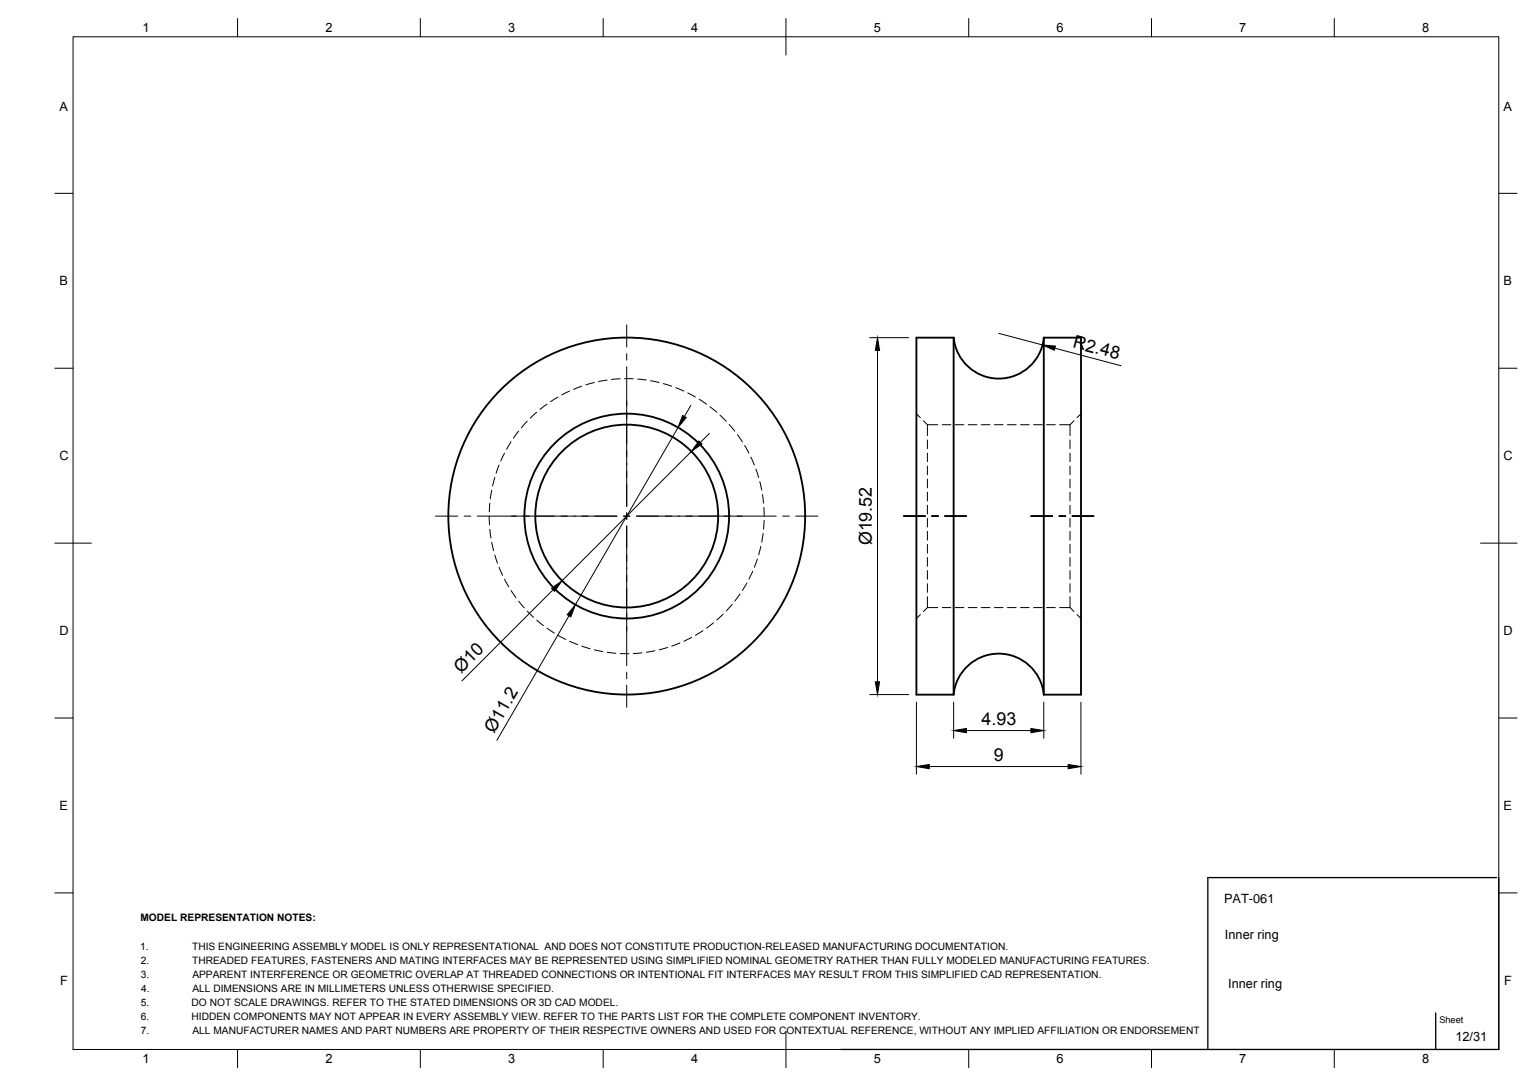
ISO-10303-21;
HEADER;
/* Generated by software containing ST-Developer
 * from STEP Tools, Inc. (www.steptools.com) 
 */

FILE_DESCRIPTION(
/* description */ ('Compact intermittent indexer'),
/* implementation_level */ '2;1');

FILE_NAME(
/* name */ 'Inner ring.step',
/* time_stamp */ '2026-10-29T16:32:17-07:00',
/* author */ (''),
/* organization */ (''),
/* preprocessor_version */ 'ST-DEVELOPER v20.2',
/* originating_system */ 'Autodesk Translation Framework v15.17.0.0',
/* authorisation */ '');

FILE_SCHEMA (('AUTOMOTIVE_DESIGN { 1 0 10303 214 3 1 1 }'));
ENDSEC;

DATA;
#10=MECHANICAL_DESIGN_GEOMETRIC_PRESENTATION_REPRESENTATION('',(#263),#10837);
#191=TOROIDAL_SURFACE('',#6190,1.,0.247676);
#199=CONICAL_SURFACE('',#6201,0.53,0.785398163397448);
#200=CONICAL_SURFACE('',#6208,0.53,0.785398163397448);
#215=SHAPE_REPRESENTATION_RELATIONSHIP('SRR','None',#10950,#239);
#239=ADVANCED_BREP_SHAPE_REPRESENTATION('',(#294),#10817);
#263=STYLED_ITEM('',(#11166),#294);
#294=MANIFOLD_SOLID_BREP('Body1',#5636);
#423=FACE_BOUND('',#1181,.T.);
#424=FACE_BOUND('',#1184,.T.);
#539=PLANE('',#6203);
#540=PLANE('',#6206);
#778=FACE_OUTER_BOUND('',#1176,.T.);
#779=FACE_OUTER_BOUND('',#1177,.T.);
#780=FACE_OUTER_BOUND('',#1178,.T.);
#781=FACE_OUTER_BOUND('',#1179,.T.);
#782=FACE_OUTER_BOUND('',#1180,.T.);
#783=FACE_OUTER_BOUND('',#1182,.T.);
#784=FACE_OUTER_BOUND('',#1183,.T.);
#785=FACE_OUTER_BOUND('',#1185,.T.);
#1176=EDGE_LOOP('',(#4228,#4229,#4230,#4231,#4232,#4233));
#1177=EDGE_LOOP('',(#4234,#4235,#4236,#4237,#4238));
#1178=EDGE_LOOP('',(#4239,#4240,#4241,#4242));
#1179=EDGE_LOOP('',(#4243,#4244,#4245,#4246));
#1180=EDGE_LOOP('',(#4247));
#1181=EDGE_LOOP('',(#4248));
#1182=EDGE_LOOP('',(#4249,#4250,#4251,#4252,#4253));
#1183=EDGE_LOOP('',(#4254));
#1184=EDGE_LOOP('',(#4255));
#1185=EDGE_LOOP('',(#4256,#4257,#4258,#4259));
#1564=LINE('',#9146,#1922);
#1565=LINE('',#9152,#1923);
#1566=LINE('',#9156,#1924);
#1567=LINE('',#9162,#1925);
#1568=LINE('',#9167,#1926);
#1922=VECTOR('',#7336,0.976185);
#1923=VECTOR('',#7343,0.5);
#1924=VECTOR('',#7348,0.53);
#1925=VECTOR('',#7357,0.976185);
#1926=VECTOR('',#7364,0.53);
#2274=CIRCLE('',#6191,0.976185);
#2275=CIRCLE('',#6192,0.976185);
#2276=CIRCLE('',#6193,0.247676);
#2277=CIRCLE('',#6194,0.976185);
#2278=CIRCLE('',#6195,0.976185);
#2279=CIRCLE('',#6197,0.976185);
#2280=CIRCLE('',#6199,0.5);
#2281=CIRCLE('',#6200,0.5);
#2282=CIRCLE('',#6202,0.56);
#2283=CIRCLE('',#6205,0.976185);
#2284=CIRCLE('',#6207,0.56);
#2654=VERTEX_POINT('',#9135);
#2655=VERTEX_POINT('',#9136);
#2656=VERTEX_POINT('',#9139);
#2657=VERTEX_POINT('',#9141);
#2658=VERTEX_POINT('',#9145);
#2659=VERTEX_POINT('',#9149);
#2660=VERTEX_POINT('',#9151);
#2661=VERTEX_POINT('',#9155);
#2662=VERTEX_POINT('',#9160);
#2663=VERTEX_POINT('',#9164);
#3236=EDGE_CURVE('',#2654,#2655,#2274,.T.);
#3237=EDGE_CURVE('',#2655,#2654,#2275,.T.);
#3238=EDGE_CURVE('',#2655,#2656,#2276,.T.);
#3239=EDGE_CURVE('',#2657,#2656,#2277,.T.);
#3240=EDGE_CURVE('',#2656,#2657,#2278,.T.);
#3241=EDGE_CURVE('',#2657,#2658,#1564,.T.);
#3242=EDGE_CURVE('',#2658,#2658,#2279,.T.);
#3243=EDGE_CURVE('',#2659,#2659,#2280,.T.);
#3244=EDGE_CURVE('',#2659,#2660,#1565,.T.);
#3245=EDGE_CURVE('',#2660,#2660,#2281,.T.);
#3246=EDGE_CURVE('',#2660,#2661,#1566,.T.);
#3247=EDGE_CURVE('',#2661,#2661,#2282,.T.);
#3248=EDGE_CURVE('',#2662,#2662,#2283,.T.);
#3249=EDGE_CURVE('',#2662,#2654,#1567,.T.);
#3250=EDGE_CURVE('',#2663,#2663,#2284,.T.);
#3251=EDGE_CURVE('',#2663,#2659,#1568,.T.);
#4228=ORIENTED_EDGE('',*,*,#3236,.F.);
#4229=ORIENTED_EDGE('',*,*,#3237,.F.);
#4230=ORIENTED_EDGE('',*,*,#3238,.T.);
#4231=ORIENTED_EDGE('',*,*,#3239,.F.);
#4232=ORIENTED_EDGE('',*,*,#3240,.F.);
#4233=ORIENTED_EDGE('',*,*,#3238,.F.);
#4234=ORIENTED_EDGE('',*,*,#3239,.T.);
#4235=ORIENTED_EDGE('',*,*,#3240,.T.);
#4236=ORIENTED_EDGE('',*,*,#3241,.T.);
#4237=ORIENTED_EDGE('',*,*,#3242,.T.);
#4238=ORIENTED_EDGE('',*,*,#3241,.F.);
#4239=ORIENTED_EDGE('',*,*,#3243,.T.);
#4240=ORIENTED_EDGE('',*,*,#3244,.T.);
#4241=ORIENTED_EDGE('',*,*,#3245,.F.);
#4242=ORIENTED_EDGE('',*,*,#3244,.F.);
#4243=ORIENTED_EDGE('',*,*,#3245,.T.);
#4244=ORIENTED_EDGE('',*,*,#3246,.T.);
#4245=ORIENTED_EDGE('',*,*,#3247,.F.);
#4246=ORIENTED_EDGE('',*,*,#3246,.F.);
#4247=ORIENTED_EDGE('',*,*,#3242,.F.);
#4248=ORIENTED_EDGE('',*,*,#3247,.T.);
#4249=ORIENTED_EDGE('',*,*,#3248,.F.);
#4250=ORIENTED_EDGE('',*,*,#3249,.T.);
#4251=ORIENTED_EDGE('',*,*,#3236,.T.);
#4252=ORIENTED_EDGE('',*,*,#3237,.T.);
#4253=ORIENTED_EDGE('',*,*,#3249,.F.);
#4254=ORIENTED_EDGE('',*,*,#3248,.T.);
#4255=ORIENTED_EDGE('',*,*,#3250,.F.);
#4256=ORIENTED_EDGE('',*,*,#3250,.T.);
#4257=ORIENTED_EDGE('',*,*,#3251,.T.);
#4258=ORIENTED_EDGE('',*,*,#3243,.F.);
#4259=ORIENTED_EDGE('',*,*,#3251,.F.);
#5226=CYLINDRICAL_SURFACE('',#6196,0.976185);
#5227=CYLINDRICAL_SURFACE('',#6198,0.5);
#5228=CYLINDRICAL_SURFACE('',#6204,0.976185);
#5421=ADVANCED_FACE('',(#778),#191,.F.);
#5422=ADVANCED_FACE('',(#779),#5226,.T.);
#5423=ADVANCED_FACE('',(#780),#5227,.F.);
#5424=ADVANCED_FACE('',(#781),#199,.F.);
#5425=ADVANCED_FACE('',(#782,#423),#539,.T.);
#5426=ADVANCED_FACE('',(#783),#5228,.T.);
#5427=ADVANCED_FACE('',(#784,#424),#540,.T.);
#5428=ADVANCED_FACE('',(#785),#200,.F.);
#5636=CLOSED_SHELL('',(#5421,#5422,#5423,#5424,#5425,#5426,#5427,#5428));
#6189=AXIS2_PLACEMENT_3D('',#9133,#7320,#7321);
#6190=AXIS2_PLACEMENT_3D('',#9134,#7322,#7323);
#6191=AXIS2_PLACEMENT_3D('',#9137,#7324,#7325);
#6192=AXIS2_PLACEMENT_3D('',#9138,#7326,#7327);
#6193=AXIS2_PLACEMENT_3D('',#9140,#7328,#7329);
#6194=AXIS2_PLACEMENT_3D('',#9142,#7330,#7331);
#6195=AXIS2_PLACEMENT_3D('',#9143,#7332,#7333);
#6196=AXIS2_PLACEMENT_3D('',#9144,#7334,#7335);
#6197=AXIS2_PLACEMENT_3D('',#9147,#7337,#7338);
#6198=AXIS2_PLACEMENT_3D('',#9148,#7339,#7340);
#6199=AXIS2_PLACEMENT_3D('',#9150,#7341,#7342);
#6200=AXIS2_PLACEMENT_3D('',#9153,#7344,#7345);
#6201=AXIS2_PLACEMENT_3D('',#9154,#7346,#7347);
#6202=AXIS2_PLACEMENT_3D('',#9157,#7349,#7350);
#6203=AXIS2_PLACEMENT_3D('',#9158,#7351,#7352);
#6204=AXIS2_PLACEMENT_3D('',#9159,#7353,#7354);
#6205=AXIS2_PLACEMENT_3D('',#9161,#7355,#7356);
#6206=AXIS2_PLACEMENT_3D('',#9163,#7358,#7359);
#6207=AXIS2_PLACEMENT_3D('',#9165,#7360,#7361);
#6208=AXIS2_PLACEMENT_3D('',#9166,#7362,#7363);
#7320=DIRECTION('axis',(0.,0.,1.));
#7321=DIRECTION('refdir',(1.,0.,0.));
#7322=DIRECTION('center_axis',(0.,-1.,0.));
#7323=DIRECTION('ref_axis',(0.,0.,-1.));
#7324=DIRECTION('center_axis',(0.,-1.,0.));
#7325=DIRECTION('ref_axis',(1.,0.,0.));
#7326=DIRECTION('center_axis',(0.,-1.,0.));
#7327=DIRECTION('ref_axis',(1.,0.,0.));
#7328=DIRECTION('center_axis',(1.,0.,1.22464679914735E-16));
#7329=DIRECTION('ref_axis',(-1.22464679914735E-16,0.,1.));
#7330=DIRECTION('center_axis',(0.,1.,0.));
#7331=DIRECTION('ref_axis',(1.,0.,0.));
#7332=DIRECTION('center_axis',(0.,1.,0.));
#7333=DIRECTION('ref_axis',(1.,0.,0.));
#7334=DIRECTION('center_axis',(0.,-1.,0.));
#7335=DIRECTION('ref_axis',(1.,0.,0.));
#7336=DIRECTION('',(0.,1.,0.));
#7337=DIRECTION('center_axis',(0.,-1.,0.));
#7338=DIRECTION('ref_axis',(1.,0.,0.));
#7339=DIRECTION('center_axis',(0.,-1.,0.));
#7340=DIRECTION('ref_axis',(1.,0.,0.));
#7341=DIRECTION('center_axis',(0.,-1.,0.));
#7342=DIRECTION('ref_axis',(1.,0.,0.));
#7343=DIRECTION('',(0.,1.,0.));
#7344=DIRECTION('center_axis',(0.,-1.,0.));
#7345=DIRECTION('ref_axis',(1.,0.,0.));
#7346=DIRECTION('center_axis',(0.,1.,0.));
#7347=DIRECTION('ref_axis',(1.,0.,0.));
#7348=DIRECTION('',(-0.707106781186547,0.707106781186548,-8.65956056235493E-17));
#7349=DIRECTION('center_axis',(0.,-1.,0.));
#7350=DIRECTION('ref_axis',(1.,0.,0.));
#7351=DIRECTION('center_axis',(0.,1.,0.));
#7352=DIRECTION('ref_axis',(0.,0.,1.));
#7353=DIRECTION('center_axis',(0.,-1.,0.));
#7354=DIRECTION('ref_axis',(1.,0.,0.));
#7355=DIRECTION('center_axis',(0.,-1.,0.));
#7356=DIRECTION('ref_axis',(1.,0.,0.));
#7357=DIRECTION('',(0.,1.,0.));
#7358=DIRECTION('center_axis',(0.,-1.,0.));
#7359=DIRECTION('ref_axis',(0.,0.,-1.));
#7360=DIRECTION('center_axis',(0.,-1.,0.));
#7361=DIRECTION('ref_axis',(1.,0.,0.));
#7362=DIRECTION('center_axis',(0.,-1.,0.));
#7363=DIRECTION('ref_axis',(1.,0.,0.));
#7364=DIRECTION('',(0.707106781186547,0.707106781186548,8.65956056235493E-17));
#9133=CARTESIAN_POINT('',(0.,0.,0.));
#9134=CARTESIAN_POINT('Origin',(0.,0.,0.));
#9135=CARTESIAN_POINT('',(-0.976185,-0.246528389340863,-1.19548183562566E-16));
#9136=CARTESIAN_POINT('',(-1.19548183562566E-16,-0.246528389340863,0.976185));
#9137=CARTESIAN_POINT('Origin',(0.,-0.246528389340863,0.));
#9138=CARTESIAN_POINT('Origin',(0.,-0.246528389340863,0.));
#9139=CARTESIAN_POINT('',(-1.19548183562566E-16,0.246528389340863,0.976185));
#9140=CARTESIAN_POINT('Origin',(-1.22464679914735E-16,0.,1.));
#9141=CARTESIAN_POINT('',(-0.976185,0.246528389340863,1.19548183562566E-16));
#9142=CARTESIAN_POINT('Origin',(0.,0.246528389340863,0.));
#9143=CARTESIAN_POINT('Origin',(0.,0.246528389340863,0.));
#9144=CARTESIAN_POINT('Origin',(0.,0.,0.));
#9145=CARTESIAN_POINT('',(-0.976185,0.45,-1.19548183562566E-16));
#9146=CARTESIAN_POINT('',(-0.976185,0.,-1.19548183562566E-16));
#9147=CARTESIAN_POINT('Origin',(0.,0.45,0.));
#9148=CARTESIAN_POINT('Origin',(0.,0.,0.));
#9149=CARTESIAN_POINT('',(-0.5,-0.39,-6.12323399573677E-17));
#9150=CARTESIAN_POINT('Origin',(0.,-0.39,0.));
#9151=CARTESIAN_POINT('',(-0.5,0.39,-6.12323399573677E-17));
#9152=CARTESIAN_POINT('',(-0.5,0.,-6.12323399573677E-17));
#9153=CARTESIAN_POINT('Origin',(0.,0.39,0.));
#9154=CARTESIAN_POINT('Origin',(0.,0.42,0.));
#9155=CARTESIAN_POINT('',(-0.56,0.45,-6.85802207522518E-17));
#9156=CARTESIAN_POINT('',(-0.53,0.42,-6.49062803548097E-17));
#9157=CARTESIAN_POINT('Origin',(0.,0.45,0.));
#9158=CARTESIAN_POINT('Origin',(0.976185,0.45,0.));
#9159=CARTESIAN_POINT('Origin',(0.,0.,0.));
#9160=CARTESIAN_POINT('',(-0.976185,-0.45,-1.19548183562566E-16));
#9161=CARTESIAN_POINT('Origin',(0.,-0.45,0.));
#9162=CARTESIAN_POINT('',(-0.976185,0.,-1.19548183562566E-16));
#9163=CARTESIAN_POINT('Origin',(0.56,-0.45,0.));
#9164=CARTESIAN_POINT('',(-0.56,-0.45,-6.85802207522518E-17));
#9165=CARTESIAN_POINT('Origin',(0.,-0.45,0.));
#9166=CARTESIAN_POINT('Origin',(0.,-0.42,0.));
#9167=CARTESIAN_POINT('',(-0.53,-0.42,-6.49062803548097E-17));
#10787=UNCERTAINTY_MEASURE_WITH_UNIT(LENGTH_MEASURE(0.001),#10838,
'DISTANCE_ACCURACY_VALUE',
'Maximum model space distance between geometric entities at asserted c
onnectivities');
#10807=UNCERTAINTY_MEASURE_WITH_UNIT(LENGTH_MEASURE(0.001),#10838,
'DISTANCE_ACCURACY_VALUE',
'Maximum model space distance between geometric entities at asserted c
onnectivities');
#10817=(
GEOMETRIC_REPRESENTATION_CONTEXT(3)
GLOBAL_UNCERTAINTY_ASSIGNED_CONTEXT((#10787))
GLOBAL_UNIT_ASSIGNED_CONTEXT((#10838,#10840,#10841))
REPRESENTATION_CONTEXT('','3D')
);
#10837=(
GEOMETRIC_REPRESENTATION_CONTEXT(3)
GLOBAL_UNCERTAINTY_ASSIGNED_CONTEXT((#10807))
GLOBAL_UNIT_ASSIGNED_CONTEXT((#10838,#10840,#10841))
REPRESENTATION_CONTEXT('','3D')
);
#10838=(
LENGTH_UNIT()
NAMED_UNIT(*)
SI_UNIT(.CENTI.,.METRE.)
);
#10840=(
NAMED_UNIT(*)
PLANE_ANGLE_UNIT()
SI_UNIT($,.RADIAN.)
);
#10841=(
NAMED_UNIT(*)
SI_UNIT($,.STERADIAN.)
SOLID_ANGLE_UNIT()
);
#10851=SHAPE_DEFINITION_REPRESENTATION(#10880,#10950);
#10880=PRODUCT_DEFINITION_SHAPE('',$,#10980);
#10950=SHAPE_REPRESENTATION('',(#6189),#10817);
#10970=PRODUCT_DEFINITION_CONTEXT('part definition',#11059,'design');
#10980=PRODUCT_DEFINITION('Inner ring','Inner ring',#11009,#10970);
#11009=PRODUCT_DEFINITION_FORMATION('',$,#11070);
#11059=APPLICATION_CONTEXT(
'Core Data for Automotive Mechanical Design Process');
#11060=PRODUCT_CONTEXT('part definition',#11059,'mechanical');
#11070=PRODUCT('Inner ring','Inner ring','Inner ring',(#11060));
#11160=COLOUR_RGB('Grey',0.48,0.52,0.57);
#11161=FILL_AREA_STYLE_COLOUR('',#11160);
#11162=FILL_AREA_STYLE('',(#11161));
#11163=SURFACE_STYLE_FILL_AREA(#11162);
#11164=SURFACE_SIDE_STYLE('',(#11163));
#11165=SURFACE_STYLE_USAGE(.BOTH.,#11164);
#11166=PRESENTATION_STYLE_ASSIGNMENT((#11165));
ENDSEC;
END-ISO-10303-21;
